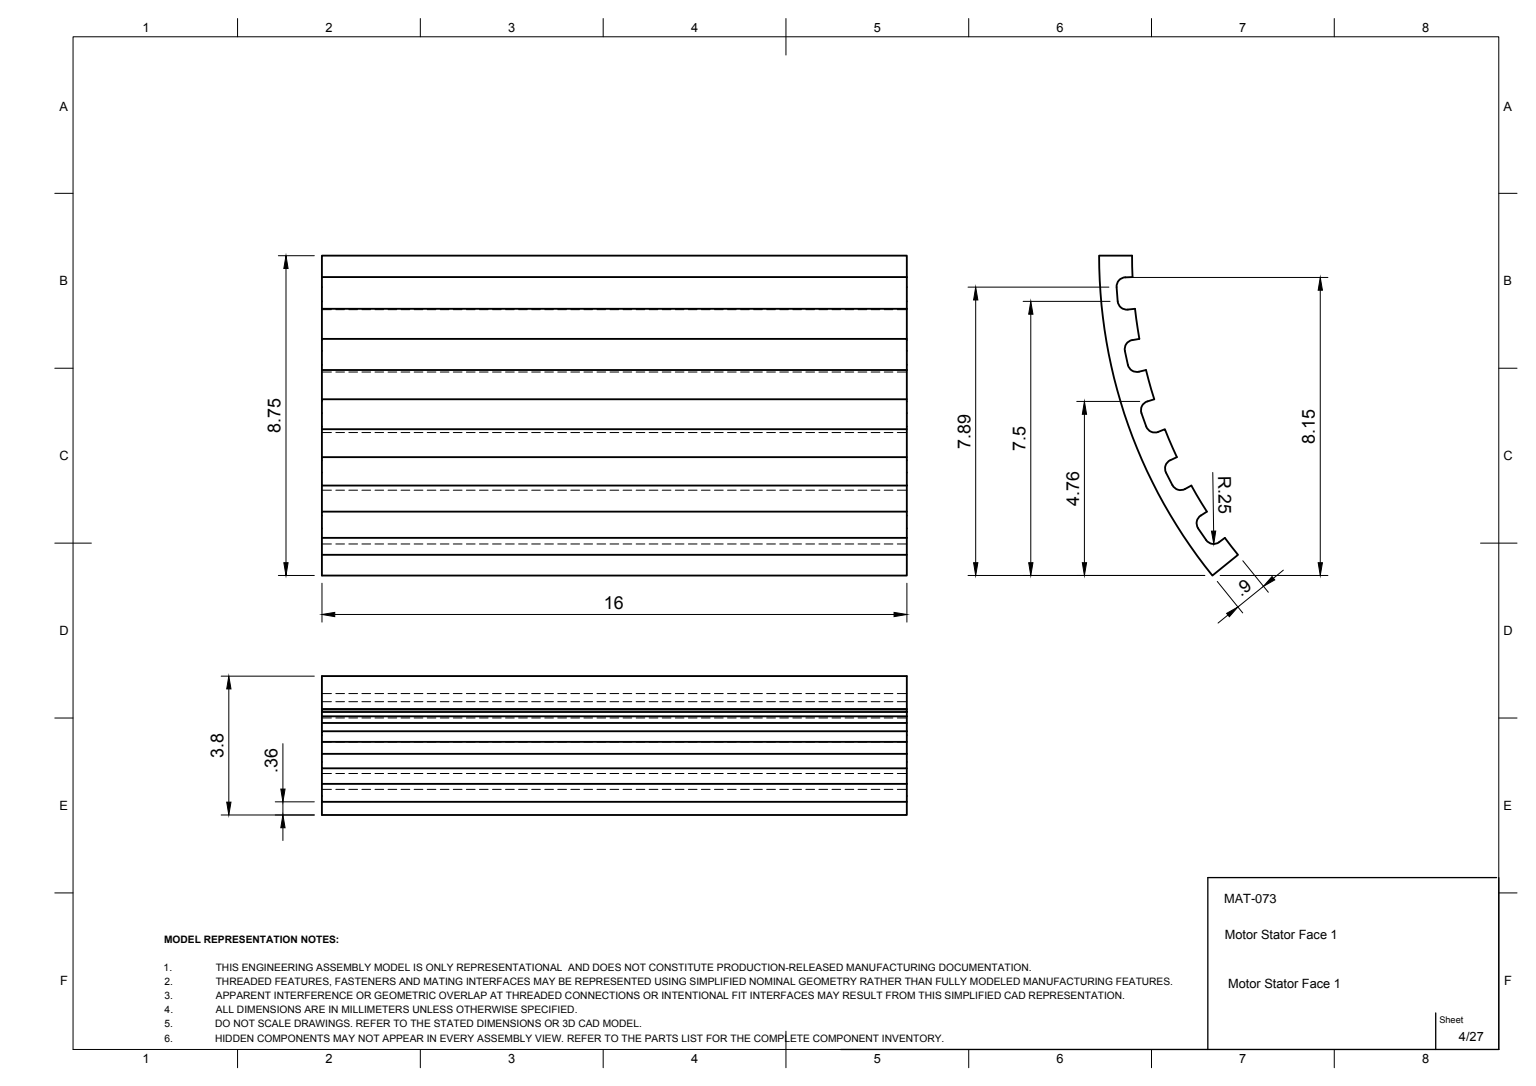
ISO-10303-21;
HEADER;
/* Generated by software containing ST-Developer
 * from STEP Tools, Inc. (www.steptools.com) 
 */

FILE_DESCRIPTION(
/* description */ ('CAx-IF Rec.Pracs.---Representation and Presentation of Product Manufa
cturing Information (PMI)---4.0---2014-10-13'),
/* implementation_level */ '2;1');

FILE_NAME(
/* name */ 'Motor Stator Face 1.step',
/* time_stamp */ '2026-10-24T18:52:33-07:00',
/* author */ (''),
/* organization */ (''),
/* preprocessor_version */ 'ST-DEVELOPER v20.2',
/* originating_system */ 'Autodesk Translation Framework v15.17.0.0',
/* authorisation */ '');

FILE_SCHEMA (('AP242_MANAGED_MODEL_BASED_3D_ENGINEERING_MIM_LF { 1 0 10303 442 2 1 4 }'));
ENDSEC;

DATA;
#10=MECHANICAL_DESIGN_GEOMETRIC_PRESENTATION_REPRESENTATION('',(#415),#34876);
#349=SHAPE_REPRESENTATION_RELATIONSHIP('SRR','None',#34986,#382);
#382=ADVANCED_BREP_SHAPE_REPRESENTATION('',(#448),#34844);
#415=STYLED_ITEM('',(#35160),#448);
#448=MANIFOLD_SOLID_BREP('Motor Stator Face 1',#19555);
#592=PLANE('',#19979);
#593=PLANE('',#19989);
#594=PLANE('',#19999);
#595=PLANE('',#20009);
#596=PLANE('',#20019);
#597=PLANE('',#20020);
#598=PLANE('',#20021);
#599=PLANE('',#20022);
#600=PLANE('',#20023);
#601=PLANE('',#20030);
#602=PLANE('',#20040);
#603=PLANE('',#20045);
#604=PLANE('',#20048);
#605=PLANE('',#20049);
#1085=LINE('',#28505,#2684);
#1086=LINE('',#28508,#2685);
#1087=LINE('',#28513,#2686);
#1088=LINE('',#28519,#2687);
#1089=LINE('',#28523,#2688);
#1090=LINE('',#28525,#2689);
#1091=LINE('',#28526,#2690);
#1092=LINE('',#28532,#2691);
#1093=LINE('',#28535,#2692);
#1094=LINE('',#28540,#2693);
#1095=LINE('',#28546,#2694);
#1096=LINE('',#28550,#2695);
#1097=LINE('',#28552,#2696);
#1098=LINE('',#28553,#2697);
#1099=LINE('',#28559,#2698);
#1100=LINE('',#28562,#2699);
#1101=LINE('',#28567,#2700);
#1102=LINE('',#28573,#2701);
#1103=LINE('',#28577,#2702);
#1104=LINE('',#28579,#2703);
#1105=LINE('',#28580,#2704);
#1106=LINE('',#28586,#2705);
#1107=LINE('',#28589,#2706);
#1108=LINE('',#28594,#2707);
#1109=LINE('',#28600,#2708);
#1110=LINE('',#28604,#2709);
#1111=LINE('',#28606,#2710);
#1112=LINE('',#28607,#2711);
#1113=LINE('',#28613,#2712);
#1114=LINE('',#28616,#2713);
#1115=LINE('',#28621,#2714);
#1116=LINE('',#28627,#2715);
#1117=LINE('',#28631,#2716);
#1118=LINE('',#28633,#2717);
#1119=LINE('',#28634,#2718);
#1120=LINE('',#28637,#2719);
#1121=LINE('',#28639,#2720);
#1122=LINE('',#28640,#2721);
#1123=LINE('',#28643,#2722);
#1124=LINE('',#28645,#2723);
#1125=LINE('',#28646,#2724);
#1126=LINE('',#28649,#2725);
#1127=LINE('',#28651,#2726);
#1128=LINE('',#28652,#2727);
#1129=LINE('',#28655,#2728);
#1130=LINE('',#28657,#2729);
#1131=LINE('',#28658,#2730);
#1132=LINE('',#28663,#2731);
#1133=LINE('',#28670,#2732);
#1134=LINE('',#28674,#2733);
#1135=LINE('',#28679,#2734);
#1136=LINE('',#28684,#2735);
#1137=LINE('',#28687,#2736);
#1138=LINE('',#28690,#2737);
#1139=LINE('',#28695,#2738);
#1140=LINE('',#28698,#2739);
#1141=LINE('',#28700,#2740);
#1142=LINE('',#28704,#2741);
#2684=VECTOR('',#22302,1.);
#2685=VECTOR('',#22305,1.);
#2686=VECTOR('',#22310,1.);
#2687=VECTOR('',#22317,1.);
#2688=VECTOR('',#22322,1.);
#2689=VECTOR('',#22323,1.);
#2690=VECTOR('',#22324,1.);
#2691=VECTOR('',#22329,1.);
#2692=VECTOR('',#22332,1.);
#2693=VECTOR('',#22337,1.);
#2694=VECTOR('',#22344,1.);
#2695=VECTOR('',#22349,0.999999999999999);
#2696=VECTOR('',#22350,1.);
#2697=VECTOR('',#22351,0.999999999999999);
#2698=VECTOR('',#22356,1.);
#2699=VECTOR('',#22359,1.);
#2700=VECTOR('',#22364,1.);
#2701=VECTOR('',#22371,1.);
#2702=VECTOR('',#22376,1.);
#2703=VECTOR('',#22377,1.);
#2704=VECTOR('',#22378,1.);
#2705=VECTOR('',#22383,1.);
#2706=VECTOR('',#22386,1.);
#2707=VECTOR('',#22391,1.);
#2708=VECTOR('',#22398,1.);
#2709=VECTOR('',#22403,1.);
#2710=VECTOR('',#22404,1.);
#2711=VECTOR('',#22405,1.);
#2712=VECTOR('',#22410,1.);
#2713=VECTOR('',#22413,1.);
#2714=VECTOR('',#22418,1.);
#2715=VECTOR('',#22425,1.);
#2716=VECTOR('',#22430,1.);
#2717=VECTOR('',#22431,1.);
#2718=VECTOR('',#22432,1.);
#2719=VECTOR('',#22435,1.);
#2720=VECTOR('',#22436,1.);
#2721=VECTOR('',#22437,1.);
#2722=VECTOR('',#22440,0.999999999999999);
#2723=VECTOR('',#22441,1.);
#2724=VECTOR('',#22442,0.999999999999999);
#2725=VECTOR('',#22445,1.);
#2726=VECTOR('',#22446,1.);
#2727=VECTOR('',#22447,1.);
#2728=VECTOR('',#22450,1.);
#2729=VECTOR('',#22451,1.);
#2730=VECTOR('',#22452,1.);
#2731=VECTOR('',#22457,1.);
#2732=VECTOR('',#22468,1.);
#2733=VECTOR('',#22471,1.);
#2734=VECTOR('',#22478,1.);
#2735=VECTOR('',#22485,1.);
#2736=VECTOR('',#22488,1.);
#2737=VECTOR('',#22493,1.);
#2738=VECTOR('',#22500,1.);
#2739=VECTOR('',#22503,1.);
#2740=VECTOR('',#22506,1.);
#2741=VECTOR('',#22513,1.);
#4283=CYLINDRICAL_SURFACE('',#19970,0.00025);
#4284=CYLINDRICAL_SURFACE('',#19973,0.01345);
#4285=CYLINDRICAL_SURFACE('',#19976,0.00025);
#4286=CYLINDRICAL_SURFACE('',#19980,0.00025);
#4287=CYLINDRICAL_SURFACE('',#19983,0.01345);
#4288=CYLINDRICAL_SURFACE('',#19986,0.00025);
#4289=CYLINDRICAL_SURFACE('',#19990,0.00025);
#4290=CYLINDRICAL_SURFACE('',#19993,0.01345);
#4291=CYLINDRICAL_SURFACE('',#19996,0.00025);
#4292=CYLINDRICAL_SURFACE('',#20000,0.00025);
#4293=CYLINDRICAL_SURFACE('',#20003,0.01345);
#4294=CYLINDRICAL_SURFACE('',#20006,0.00025);
#4295=CYLINDRICAL_SURFACE('',#20010,0.00025);
#4296=CYLINDRICAL_SURFACE('',#20013,0.01345);
#4297=CYLINDRICAL_SURFACE('',#20016,0.00025);
#4298=CYLINDRICAL_SURFACE('',#20024,0.013);
#4299=CYLINDRICAL_SURFACE('',#20027,0.013);
#4300=CYLINDRICAL_SURFACE('',#20036,0.013);
#4301=CYLINDRICAL_SURFACE('',#20038,0.013);
#4302=CYLINDRICAL_SURFACE('',#20041,0.013);
#4303=CYLINDRICAL_SURFACE('',#20043,0.0139);
#4304=CYLINDRICAL_SURFACE('',#20046,0.013);
#4799=FACE_OUTER_BOUND('',#5846,.T.);
#4800=FACE_OUTER_BOUND('',#5847,.T.);
#4801=FACE_OUTER_BOUND('',#5848,.T.);
#4802=FACE_OUTER_BOUND('',#5849,.T.);
#4803=FACE_OUTER_BOUND('',#5850,.T.);
#4804=FACE_OUTER_BOUND('',#5851,.T.);
#4805=FACE_OUTER_BOUND('',#5852,.T.);
#4806=FACE_OUTER_BOUND('',#5853,.T.);
#4807=FACE_OUTER_BOUND('',#5854,.T.);
#4808=FACE_OUTER_BOUND('',#5855,.T.);
#4809=FACE_OUTER_BOUND('',#5856,.T.);
#4810=FACE_OUTER_BOUND('',#5857,.T.);
#4811=FACE_OUTER_BOUND('',#5858,.T.);
#4812=FACE_OUTER_BOUND('',#5859,.T.);
#4813=FACE_OUTER_BOUND('',#5860,.T.);
#4814=FACE_OUTER_BOUND('',#5861,.T.);
#4815=FACE_OUTER_BOUND('',#5862,.T.);
#4816=FACE_OUTER_BOUND('',#5863,.T.);
#4817=FACE_OUTER_BOUND('',#5864,.T.);
#4818=FACE_OUTER_BOUND('',#5865,.T.);
#4819=FACE_OUTER_BOUND('',#5866,.T.);
#4820=FACE_OUTER_BOUND('',#5867,.T.);
#4821=FACE_OUTER_BOUND('',#5868,.T.);
#4822=FACE_OUTER_BOUND('',#5869,.T.);
#4823=FACE_OUTER_BOUND('',#5870,.T.);
#4824=FACE_OUTER_BOUND('',#5871,.T.);
#4825=FACE_OUTER_BOUND('',#5872,.T.);
#4826=FACE_OUTER_BOUND('',#5873,.T.);
#4827=FACE_OUTER_BOUND('',#5874,.T.);
#4828=FACE_OUTER_BOUND('',#5875,.T.);
#4829=FACE_OUTER_BOUND('',#5876,.T.);
#4830=FACE_OUTER_BOUND('',#5877,.T.);
#4831=FACE_OUTER_BOUND('',#5878,.T.);
#4832=FACE_OUTER_BOUND('',#5879,.T.);
#4833=FACE_OUTER_BOUND('',#5880,.T.);
#4834=FACE_OUTER_BOUND('',#5881,.T.);
#5846=EDGE_LOOP('',(#12830,#12831,#12832,#12833));
#5847=EDGE_LOOP('',(#12834,#12835,#12836,#12837));
#5848=EDGE_LOOP('',(#12838,#12839,#12840,#12841));
#5849=EDGE_LOOP('',(#12842,#12843,#12844,#12845));
#5850=EDGE_LOOP('',(#12846,#12847,#12848,#12849));
#5851=EDGE_LOOP('',(#12850,#12851,#12852,#12853));
#5852=EDGE_LOOP('',(#12854,#12855,#12856,#12857));
#5853=EDGE_LOOP('',(#12858,#12859,#12860,#12861));
#5854=EDGE_LOOP('',(#12862,#12863,#12864,#12865));
#5855=EDGE_LOOP('',(#12866,#12867,#12868,#12869));
#5856=EDGE_LOOP('',(#12870,#12871,#12872,#12873));
#5857=EDGE_LOOP('',(#12874,#12875,#12876,#12877));
#5858=EDGE_LOOP('',(#12878,#12879,#12880,#12881));
#5859=EDGE_LOOP('',(#12882,#12883,#12884,#12885));
#5860=EDGE_LOOP('',(#12886,#12887,#12888,#12889));
#5861=EDGE_LOOP('',(#12890,#12891,#12892,#12893));
#5862=EDGE_LOOP('',(#12894,#12895,#12896,#12897));
#5863=EDGE_LOOP('',(#12898,#12899,#12900,#12901));
#5864=EDGE_LOOP('',(#12902,#12903,#12904,#12905));
#5865=EDGE_LOOP('',(#12906,#12907,#12908,#12909));
#5866=EDGE_LOOP('',(#12910,#12911,#12912,#12913));
#5867=EDGE_LOOP('',(#12914,#12915,#12916,#12917));
#5868=EDGE_LOOP('',(#12918,#12919,#12920,#12921));
#5869=EDGE_LOOP('',(#12922,#12923,#12924,#12925));
#5870=EDGE_LOOP('',(#12926,#12927,#12928,#12929));
#5871=EDGE_LOOP('',(#12930,#12931,#12932,#12933));
#5872=EDGE_LOOP('',(#12934,#12935,#12936,#12937,#12938,#12939,#12940,#12941,
#12942,#12943,#12944,#12945,#12946,#12947,#12948,#12949,#12950,#12951,#12952,
#12953,#12954,#12955,#12956,#12957,#12958,#12959,#12960,#12961,#12962,#12963,
#12964,#12965,#12966,#12967));
#5873=EDGE_LOOP('',(#12968,#12969,#12970,#12971));
#5874=EDGE_LOOP('',(#12972,#12973,#12974,#12975));
#5875=EDGE_LOOP('',(#12976,#12977,#12978,#12979));
#5876=EDGE_LOOP('',(#12980,#12981,#12982,#12983));
#5877=EDGE_LOOP('',(#12984,#12985,#12986,#12987));
#5878=EDGE_LOOP('',(#12988,#12989,#12990,#12991));
#5879=EDGE_LOOP('',(#12992,#12993,#12994,#12995));
#5880=EDGE_LOOP('',(#12996,#12997,#12998,#12999));
#5881=EDGE_LOOP('',(#13000,#13001,#13002,#13003,#13004,#13005,#13006,#13007,
#13008,#13009,#13010,#13011,#13012,#13013,#13014,#13015,#13016,#13017,#13018,
#13019,#13020,#13021,#13022,#13023,#13024,#13025,#13026,#13027,#13028,#13029,
#13030,#13031,#13032,#13033));
#7003=CIRCLE('',#19971,0.000250000000012414);
#7004=CIRCLE('',#19972,0.000250000000012414);
#7005=CIRCLE('',#19974,0.0134500000000135);
#7006=CIRCLE('',#19975,0.0134500000000135);
#7007=CIRCLE('',#19977,0.000250000000012074);
#7008=CIRCLE('',#19978,0.000250000000012074);
#7009=CIRCLE('',#19981,0.000250000000011423);
#7010=CIRCLE('',#19982,0.000250000000011423);
#7011=CIRCLE('',#19984,0.0134500000000139);
#7012=CIRCLE('',#19985,0.0134500000000139);
#7013=CIRCLE('',#19987,0.00025000000001101);
#7014=CIRCLE('',#19988,0.00025000000001101);
#7015=CIRCLE('',#19991,0.000250000000010237);
#7016=CIRCLE('',#19992,0.000250000000010237);
#7017=CIRCLE('',#19994,0.0134500000000141);
#7018=CIRCLE('',#19995,0.0134500000000141);
#7019=CIRCLE('',#19997,0.000250000000010237);
#7020=CIRCLE('',#19998,0.000250000000010237);
#7021=CIRCLE('',#20001,0.00025000000001101);
#7022=CIRCLE('',#20002,0.00025000000001101);
#7023=CIRCLE('',#20004,0.0134500000000141);
#7024=CIRCLE('',#20005,0.0134500000000141);
#7025=CIRCLE('',#20007,0.000250000000011423);
#7026=CIRCLE('',#20008,0.000250000000011423);
#7027=CIRCLE('',#20011,0.000250000000012074);
#7028=CIRCLE('',#20012,0.000250000000012074);
#7029=CIRCLE('',#20014,0.0134500000000138);
#7030=CIRCLE('',#20015,0.0134500000000138);
#7031=CIRCLE('',#20017,0.000250000000012414);
#7032=CIRCLE('',#20018,0.000250000000012414);
#7033=CIRCLE('',#20025,0.0130000000000133);
#7034=CIRCLE('',#20026,0.0130000000000133);
#7035=CIRCLE('',#20028,0.0130000000000133);
#7036=CIRCLE('',#20029,0.0130000000000133);
#7037=CIRCLE('',#20031,0.0139000000000133);
#7038=CIRCLE('',#20032,0.0130000000000133);
#7039=CIRCLE('',#20033,0.0130000000000133);
#7040=CIRCLE('',#20034,0.0130000000000133);
#7041=CIRCLE('',#20035,0.0130000000000133);
#7042=CIRCLE('',#20037,0.0130000000000133);
#7043=CIRCLE('',#20039,0.0130000000000133);
#7044=CIRCLE('',#20042,0.0130000000000133);
#7045=CIRCLE('',#20044,0.0139000000000133);
#7046=CIRCLE('',#20047,0.0130000000000133);
#8081=VERTEX_POINT('',#28501);
#8082=VERTEX_POINT('',#28502);
#8083=VERTEX_POINT('',#28504);
#8084=VERTEX_POINT('',#28506);
#8085=VERTEX_POINT('',#28510);
#8086=VERTEX_POINT('',#28512);
#8087=VERTEX_POINT('',#28516);
#8088=VERTEX_POINT('',#28518);
#8089=VERTEX_POINT('',#28522);
#8090=VERTEX_POINT('',#28524);
#8091=VERTEX_POINT('',#28528);
#8092=VERTEX_POINT('',#28529);
#8093=VERTEX_POINT('',#28531);
#8094=VERTEX_POINT('',#28533);
#8095=VERTEX_POINT('',#28537);
#8096=VERTEX_POINT('',#28539);
#8097=VERTEX_POINT('',#28543);
#8098=VERTEX_POINT('',#28545);
#8099=VERTEX_POINT('',#28549);
#8100=VERTEX_POINT('',#28551);
#8101=VERTEX_POINT('',#28555);
#8102=VERTEX_POINT('',#28556);
#8103=VERTEX_POINT('',#28558);
#8104=VERTEX_POINT('',#28560);
#8105=VERTEX_POINT('',#28564);
#8106=VERTEX_POINT('',#28566);
#8107=VERTEX_POINT('',#28570);
#8108=VERTEX_POINT('',#28572);
#8109=VERTEX_POINT('',#28576);
#8110=VERTEX_POINT('',#28578);
#8111=VERTEX_POINT('',#28582);
#8112=VERTEX_POINT('',#28583);
#8113=VERTEX_POINT('',#28585);
#8114=VERTEX_POINT('',#28587);
#8115=VERTEX_POINT('',#28591);
#8116=VERTEX_POINT('',#28593);
#8117=VERTEX_POINT('',#28597);
#8118=VERTEX_POINT('',#28599);
#8119=VERTEX_POINT('',#28603);
#8120=VERTEX_POINT('',#28605);
#8121=VERTEX_POINT('',#28609);
#8122=VERTEX_POINT('',#28610);
#8123=VERTEX_POINT('',#28612);
#8124=VERTEX_POINT('',#28614);
#8125=VERTEX_POINT('',#28618);
#8126=VERTEX_POINT('',#28620);
#8127=VERTEX_POINT('',#28624);
#8128=VERTEX_POINT('',#28626);
#8129=VERTEX_POINT('',#28630);
#8130=VERTEX_POINT('',#28632);
#8131=VERTEX_POINT('',#28636);
#8132=VERTEX_POINT('',#28638);
#8133=VERTEX_POINT('',#28642);
#8134=VERTEX_POINT('',#28644);
#8135=VERTEX_POINT('',#28648);
#8136=VERTEX_POINT('',#28650);
#8137=VERTEX_POINT('',#28654);
#8138=VERTEX_POINT('',#28656);
#8139=VERTEX_POINT('',#28660);
#8140=VERTEX_POINT('',#28662);
#8141=VERTEX_POINT('',#28669);
#8142=VERTEX_POINT('',#28671);
#8143=VERTEX_POINT('',#28673);
#8144=VERTEX_POINT('',#28677);
#8145=VERTEX_POINT('',#28682);
#8146=VERTEX_POINT('',#28686);
#8147=VERTEX_POINT('',#28694);
#8148=VERTEX_POINT('',#28696);
#9973=EDGE_CURVE('',#8081,#8082,#7003,.T.);
#9974=EDGE_CURVE('',#8082,#8083,#1085,.T.);
#9975=EDGE_CURVE('',#8083,#8084,#7004,.T.);
#9976=EDGE_CURVE('',#8084,#8081,#1086,.T.);
#9977=EDGE_CURVE('',#8085,#8082,#7005,.T.);
#9978=EDGE_CURVE('',#8086,#8085,#1087,.T.);
#9979=EDGE_CURVE('',#8083,#8086,#7006,.T.);
#9980=EDGE_CURVE('',#8085,#8087,#7007,.T.);
#9981=EDGE_CURVE('',#8087,#8088,#1088,.T.);
#9982=EDGE_CURVE('',#8088,#8086,#7008,.T.);
#9983=EDGE_CURVE('',#8089,#8087,#1089,.T.);
#9984=EDGE_CURVE('',#8090,#8089,#1090,.T.);
#9985=EDGE_CURVE('',#8088,#8090,#1091,.T.);
#9986=EDGE_CURVE('',#8091,#8092,#7009,.T.);
#9987=EDGE_CURVE('',#8092,#8093,#1092,.T.);
#9988=EDGE_CURVE('',#8093,#8094,#7010,.T.);
#9989=EDGE_CURVE('',#8094,#8091,#1093,.T.);
#9990=EDGE_CURVE('',#8095,#8092,#7011,.T.);
#9991=EDGE_CURVE('',#8096,#8095,#1094,.T.);
#9992=EDGE_CURVE('',#8093,#8096,#7012,.T.);
#9993=EDGE_CURVE('',#8095,#8097,#7013,.T.);
#9994=EDGE_CURVE('',#8097,#8098,#1095,.T.);
#9995=EDGE_CURVE('',#8098,#8096,#7014,.T.);
#9996=EDGE_CURVE('',#8099,#8097,#1096,.T.);
#9997=EDGE_CURVE('',#8100,#8099,#1097,.T.);
#9998=EDGE_CURVE('',#8098,#8100,#1098,.T.);
#9999=EDGE_CURVE('',#8101,#8102,#7015,.T.);
#10000=EDGE_CURVE('',#8102,#8103,#1099,.T.);
#10001=EDGE_CURVE('',#8103,#8104,#7016,.T.);
#10002=EDGE_CURVE('',#8104,#8101,#1100,.T.);
#10003=EDGE_CURVE('',#8105,#8102,#7017,.T.);
#10004=EDGE_CURVE('',#8106,#8105,#1101,.T.);
#10005=EDGE_CURVE('',#8103,#8106,#7018,.T.);
#10006=EDGE_CURVE('',#8105,#8107,#7019,.T.);
#10007=EDGE_CURVE('',#8107,#8108,#1102,.T.);
#10008=EDGE_CURVE('',#8108,#8106,#7020,.T.);
#10009=EDGE_CURVE('',#8109,#8107,#1103,.T.);
#10010=EDGE_CURVE('',#8110,#8109,#1104,.T.);
#10011=EDGE_CURVE('',#8108,#8110,#1105,.T.);
#10012=EDGE_CURVE('',#8111,#8112,#7021,.T.);
#10013=EDGE_CURVE('',#8112,#8113,#1106,.T.);
#10014=EDGE_CURVE('',#8113,#8114,#7022,.T.);
#10015=EDGE_CURVE('',#8114,#8111,#1107,.T.);
#10016=EDGE_CURVE('',#8115,#8112,#7023,.T.);
#10017=EDGE_CURVE('',#8116,#8115,#1108,.T.);
#10018=EDGE_CURVE('',#8113,#8116,#7024,.T.);
#10019=EDGE_CURVE('',#8115,#8117,#7025,.T.);
#10020=EDGE_CURVE('',#8117,#8118,#1109,.T.);
#10021=EDGE_CURVE('',#8118,#8116,#7026,.T.);
#10022=EDGE_CURVE('',#8119,#8117,#1110,.T.);
#10023=EDGE_CURVE('',#8120,#8119,#1111,.T.);
#10024=EDGE_CURVE('',#8118,#8120,#1112,.T.);
#10025=EDGE_CURVE('',#8121,#8122,#7027,.T.);
#10026=EDGE_CURVE('',#8122,#8123,#1113,.T.);
#10027=EDGE_CURVE('',#8123,#8124,#7028,.T.);
#10028=EDGE_CURVE('',#8124,#8121,#1114,.T.);
#10029=EDGE_CURVE('',#8125,#8122,#7029,.T.);
#10030=EDGE_CURVE('',#8126,#8125,#1115,.T.);
#10031=EDGE_CURVE('',#8123,#8126,#7030,.T.);
#10032=EDGE_CURVE('',#8125,#8127,#7031,.T.);
#10033=EDGE_CURVE('',#8127,#8128,#1116,.T.);
#10034=EDGE_CURVE('',#8128,#8126,#7032,.T.);
#10035=EDGE_CURVE('',#8129,#8127,#1117,.T.);
#10036=EDGE_CURVE('',#8130,#8129,#1118,.T.);
#10037=EDGE_CURVE('',#8128,#8130,#1119,.T.);
#10038=EDGE_CURVE('',#8131,#8124,#1120,.T.);
#10039=EDGE_CURVE('',#8132,#8131,#1121,.T.);
#10040=EDGE_CURVE('',#8121,#8132,#1122,.T.);
#10041=EDGE_CURVE('',#8133,#8114,#1123,.T.);
#10042=EDGE_CURVE('',#8134,#8133,#1124,.T.);
#10043=EDGE_CURVE('',#8111,#8134,#1125,.T.);
#10044=EDGE_CURVE('',#8135,#8094,#1126,.T.);
#10045=EDGE_CURVE('',#8136,#8135,#1127,.T.);
#10046=EDGE_CURVE('',#8091,#8136,#1128,.T.);
#10047=EDGE_CURVE('',#8137,#8084,#1129,.T.);
#10048=EDGE_CURVE('',#8138,#8137,#1130,.T.);
#10049=EDGE_CURVE('',#8081,#8138,#1131,.T.);
#10050=EDGE_CURVE('',#8139,#8129,#7033,.T.);
#10051=EDGE_CURVE('',#8140,#8139,#1132,.T.);
#10052=EDGE_CURVE('',#8130,#8140,#7034,.T.);
#10053=EDGE_CURVE('',#8110,#8133,#7035,.T.);
#10054=EDGE_CURVE('',#8134,#8109,#7036,.T.);
#10055=EDGE_CURVE('',#8140,#8141,#1133,.T.);
#10056=EDGE_CURVE('',#8141,#8142,#7037,.T.);
#10057=EDGE_CURVE('',#8142,#8143,#1134,.T.);
#10058=EDGE_CURVE('',#8143,#8137,#7038,.T.);
#10059=EDGE_CURVE('',#8090,#8135,#7039,.T.);
#10060=EDGE_CURVE('',#8100,#8144,#7040,.T.);
#10061=EDGE_CURVE('',#8144,#8104,#1135,.T.);
#10062=EDGE_CURVE('',#8120,#8131,#7041,.T.);
#10063=EDGE_CURVE('',#8145,#8099,#7042,.T.);
#10064=EDGE_CURVE('',#8145,#8144,#1136,.T.);
#10065=EDGE_CURVE('',#8143,#8146,#1137,.T.);
#10066=EDGE_CURVE('',#8138,#8146,#7043,.T.);
#10067=EDGE_CURVE('',#8101,#8145,#1138,.T.);
#10068=EDGE_CURVE('',#8132,#8119,#7044,.T.);
#10069=EDGE_CURVE('',#8147,#8141,#1139,.T.);
#10070=EDGE_CURVE('',#8148,#8147,#7045,.T.);
#10071=EDGE_CURVE('',#8142,#8148,#1140,.T.);
#10072=EDGE_CURVE('',#8146,#8148,#1141,.T.);
#10073=EDGE_CURVE('',#8136,#8089,#7046,.T.);
#10074=EDGE_CURVE('',#8147,#8139,#1142,.T.);
#12830=ORIENTED_EDGE('',*,*,#9973,.T.);
#12831=ORIENTED_EDGE('',*,*,#9974,.T.);
#12832=ORIENTED_EDGE('',*,*,#9975,.T.);
#12833=ORIENTED_EDGE('',*,*,#9976,.T.);
#12834=ORIENTED_EDGE('',*,*,#9974,.F.);
#12835=ORIENTED_EDGE('',*,*,#9977,.F.);
#12836=ORIENTED_EDGE('',*,*,#9978,.F.);
#12837=ORIENTED_EDGE('',*,*,#9979,.F.);
#12838=ORIENTED_EDGE('',*,*,#9980,.T.);
#12839=ORIENTED_EDGE('',*,*,#9981,.T.);
#12840=ORIENTED_EDGE('',*,*,#9982,.T.);
#12841=ORIENTED_EDGE('',*,*,#9978,.T.);
#12842=ORIENTED_EDGE('',*,*,#9981,.F.);
#12843=ORIENTED_EDGE('',*,*,#9983,.F.);
#12844=ORIENTED_EDGE('',*,*,#9984,.F.);
#12845=ORIENTED_EDGE('',*,*,#9985,.F.);
#12846=ORIENTED_EDGE('',*,*,#9986,.T.);
#12847=ORIENTED_EDGE('',*,*,#9987,.T.);
#12848=ORIENTED_EDGE('',*,*,#9988,.T.);
#12849=ORIENTED_EDGE('',*,*,#9989,.T.);
#12850=ORIENTED_EDGE('',*,*,#9987,.F.);
#12851=ORIENTED_EDGE('',*,*,#9990,.F.);
#12852=ORIENTED_EDGE('',*,*,#9991,.F.);
#12853=ORIENTED_EDGE('',*,*,#9992,.F.);
#12854=ORIENTED_EDGE('',*,*,#9993,.T.);
#12855=ORIENTED_EDGE('',*,*,#9994,.T.);
#12856=ORIENTED_EDGE('',*,*,#9995,.T.);
#12857=ORIENTED_EDGE('',*,*,#9991,.T.);
#12858=ORIENTED_EDGE('',*,*,#9994,.F.);
#12859=ORIENTED_EDGE('',*,*,#9996,.F.);
#12860=ORIENTED_EDGE('',*,*,#9997,.F.);
#12861=ORIENTED_EDGE('',*,*,#9998,.F.);
#12862=ORIENTED_EDGE('',*,*,#9999,.T.);
#12863=ORIENTED_EDGE('',*,*,#10000,.T.);
#12864=ORIENTED_EDGE('',*,*,#10001,.T.);
#12865=ORIENTED_EDGE('',*,*,#10002,.T.);
#12866=ORIENTED_EDGE('',*,*,#10000,.F.);
#12867=ORIENTED_EDGE('',*,*,#10003,.F.);
#12868=ORIENTED_EDGE('',*,*,#10004,.F.);
#12869=ORIENTED_EDGE('',*,*,#10005,.F.);
#12870=ORIENTED_EDGE('',*,*,#10006,.T.);
#12871=ORIENTED_EDGE('',*,*,#10007,.T.);
#12872=ORIENTED_EDGE('',*,*,#10008,.T.);
#12873=ORIENTED_EDGE('',*,*,#10004,.T.);
#12874=ORIENTED_EDGE('',*,*,#10007,.F.);
#12875=ORIENTED_EDGE('',*,*,#10009,.F.);
#12876=ORIENTED_EDGE('',*,*,#10010,.F.);
#12877=ORIENTED_EDGE('',*,*,#10011,.F.);
#12878=ORIENTED_EDGE('',*,*,#10012,.T.);
#12879=ORIENTED_EDGE('',*,*,#10013,.T.);
#12880=ORIENTED_EDGE('',*,*,#10014,.T.);
#12881=ORIENTED_EDGE('',*,*,#10015,.T.);
#12882=ORIENTED_EDGE('',*,*,#10013,.F.);
#12883=ORIENTED_EDGE('',*,*,#10016,.F.);
#12884=ORIENTED_EDGE('',*,*,#10017,.F.);
#12885=ORIENTED_EDGE('',*,*,#10018,.F.);
#12886=ORIENTED_EDGE('',*,*,#10019,.T.);
#12887=ORIENTED_EDGE('',*,*,#10020,.T.);
#12888=ORIENTED_EDGE('',*,*,#10021,.T.);
#12889=ORIENTED_EDGE('',*,*,#10017,.T.);
#12890=ORIENTED_EDGE('',*,*,#10020,.F.);
#12891=ORIENTED_EDGE('',*,*,#10022,.F.);
#12892=ORIENTED_EDGE('',*,*,#10023,.F.);
#12893=ORIENTED_EDGE('',*,*,#10024,.F.);
#12894=ORIENTED_EDGE('',*,*,#10025,.T.);
#12895=ORIENTED_EDGE('',*,*,#10026,.T.);
#12896=ORIENTED_EDGE('',*,*,#10027,.T.);
#12897=ORIENTED_EDGE('',*,*,#10028,.T.);
#12898=ORIENTED_EDGE('',*,*,#10026,.F.);
#12899=ORIENTED_EDGE('',*,*,#10029,.F.);
#12900=ORIENTED_EDGE('',*,*,#10030,.F.);
#12901=ORIENTED_EDGE('',*,*,#10031,.F.);
#12902=ORIENTED_EDGE('',*,*,#10032,.T.);
#12903=ORIENTED_EDGE('',*,*,#10033,.T.);
#12904=ORIENTED_EDGE('',*,*,#10034,.T.);
#12905=ORIENTED_EDGE('',*,*,#10030,.T.);
#12906=ORIENTED_EDGE('',*,*,#10033,.F.);
#12907=ORIENTED_EDGE('',*,*,#10035,.F.);
#12908=ORIENTED_EDGE('',*,*,#10036,.F.);
#12909=ORIENTED_EDGE('',*,*,#10037,.F.);
#12910=ORIENTED_EDGE('',*,*,#10028,.F.);
#12911=ORIENTED_EDGE('',*,*,#10038,.F.);
#12912=ORIENTED_EDGE('',*,*,#10039,.F.);
#12913=ORIENTED_EDGE('',*,*,#10040,.F.);
#12914=ORIENTED_EDGE('',*,*,#10015,.F.);
#12915=ORIENTED_EDGE('',*,*,#10041,.F.);
#12916=ORIENTED_EDGE('',*,*,#10042,.F.);
#12917=ORIENTED_EDGE('',*,*,#10043,.F.);
#12918=ORIENTED_EDGE('',*,*,#9989,.F.);
#12919=ORIENTED_EDGE('',*,*,#10044,.F.);
#12920=ORIENTED_EDGE('',*,*,#10045,.F.);
#12921=ORIENTED_EDGE('',*,*,#10046,.F.);
#12922=ORIENTED_EDGE('',*,*,#9976,.F.);
#12923=ORIENTED_EDGE('',*,*,#10047,.F.);
#12924=ORIENTED_EDGE('',*,*,#10048,.F.);
#12925=ORIENTED_EDGE('',*,*,#10049,.F.);
#12926=ORIENTED_EDGE('',*,*,#10036,.T.);
#12927=ORIENTED_EDGE('',*,*,#10050,.F.);
#12928=ORIENTED_EDGE('',*,*,#10051,.F.);
#12929=ORIENTED_EDGE('',*,*,#10052,.F.);
#12930=ORIENTED_EDGE('',*,*,#10042,.T.);
#12931=ORIENTED_EDGE('',*,*,#10053,.F.);
#12932=ORIENTED_EDGE('',*,*,#10010,.T.);
#12933=ORIENTED_EDGE('',*,*,#10054,.F.);
#12934=ORIENTED_EDGE('',*,*,#10038,.T.);
#12935=ORIENTED_EDGE('',*,*,#10027,.F.);
#12936=ORIENTED_EDGE('',*,*,#10031,.T.);
#12937=ORIENTED_EDGE('',*,*,#10034,.F.);
#12938=ORIENTED_EDGE('',*,*,#10037,.T.);
#12939=ORIENTED_EDGE('',*,*,#10052,.T.);
#12940=ORIENTED_EDGE('',*,*,#10055,.T.);
#12941=ORIENTED_EDGE('',*,*,#10056,.T.);
#12942=ORIENTED_EDGE('',*,*,#10057,.T.);
#12943=ORIENTED_EDGE('',*,*,#10058,.T.);
#12944=ORIENTED_EDGE('',*,*,#10047,.T.);
#12945=ORIENTED_EDGE('',*,*,#9975,.F.);
#12946=ORIENTED_EDGE('',*,*,#9979,.T.);
#12947=ORIENTED_EDGE('',*,*,#9982,.F.);
#12948=ORIENTED_EDGE('',*,*,#9985,.T.);
#12949=ORIENTED_EDGE('',*,*,#10059,.T.);
#12950=ORIENTED_EDGE('',*,*,#10044,.T.);
#12951=ORIENTED_EDGE('',*,*,#9988,.F.);
#12952=ORIENTED_EDGE('',*,*,#9992,.T.);
#12953=ORIENTED_EDGE('',*,*,#9995,.F.);
#12954=ORIENTED_EDGE('',*,*,#9998,.T.);
#12955=ORIENTED_EDGE('',*,*,#10060,.T.);
#12956=ORIENTED_EDGE('',*,*,#10061,.T.);
#12957=ORIENTED_EDGE('',*,*,#10001,.F.);
#12958=ORIENTED_EDGE('',*,*,#10005,.T.);
#12959=ORIENTED_EDGE('',*,*,#10008,.F.);
#12960=ORIENTED_EDGE('',*,*,#10011,.T.);
#12961=ORIENTED_EDGE('',*,*,#10053,.T.);
#12962=ORIENTED_EDGE('',*,*,#10041,.T.);
#12963=ORIENTED_EDGE('',*,*,#10014,.F.);
#12964=ORIENTED_EDGE('',*,*,#10018,.T.);
#12965=ORIENTED_EDGE('',*,*,#10021,.F.);
#12966=ORIENTED_EDGE('',*,*,#10024,.T.);
#12967=ORIENTED_EDGE('',*,*,#10062,.T.);
#12968=ORIENTED_EDGE('',*,*,#9997,.T.);
#12969=ORIENTED_EDGE('',*,*,#10063,.F.);
#12970=ORIENTED_EDGE('',*,*,#10064,.T.);
#12971=ORIENTED_EDGE('',*,*,#10060,.F.);
#12972=ORIENTED_EDGE('',*,*,#10048,.T.);
#12973=ORIENTED_EDGE('',*,*,#10058,.F.);
#12974=ORIENTED_EDGE('',*,*,#10065,.T.);
#12975=ORIENTED_EDGE('',*,*,#10066,.F.);
#12976=ORIENTED_EDGE('',*,*,#10002,.F.);
#12977=ORIENTED_EDGE('',*,*,#10061,.F.);
#12978=ORIENTED_EDGE('',*,*,#10064,.F.);
#12979=ORIENTED_EDGE('',*,*,#10067,.F.);
#12980=ORIENTED_EDGE('',*,*,#10039,.T.);
#12981=ORIENTED_EDGE('',*,*,#10062,.F.);
#12982=ORIENTED_EDGE('',*,*,#10023,.T.);
#12983=ORIENTED_EDGE('',*,*,#10068,.F.);
#12984=ORIENTED_EDGE('',*,*,#10069,.F.);
#12985=ORIENTED_EDGE('',*,*,#10070,.F.);
#12986=ORIENTED_EDGE('',*,*,#10071,.F.);
#12987=ORIENTED_EDGE('',*,*,#10056,.F.);
#12988=ORIENTED_EDGE('',*,*,#10071,.T.);
#12989=ORIENTED_EDGE('',*,*,#10072,.F.);
#12990=ORIENTED_EDGE('',*,*,#10065,.F.);
#12991=ORIENTED_EDGE('',*,*,#10057,.F.);
#12992=ORIENTED_EDGE('',*,*,#10045,.T.);
#12993=ORIENTED_EDGE('',*,*,#10059,.F.);
#12994=ORIENTED_EDGE('',*,*,#9984,.T.);
#12995=ORIENTED_EDGE('',*,*,#10073,.F.);
#12996=ORIENTED_EDGE('',*,*,#10051,.T.);
#12997=ORIENTED_EDGE('',*,*,#10074,.F.);
#12998=ORIENTED_EDGE('',*,*,#10069,.T.);
#12999=ORIENTED_EDGE('',*,*,#10055,.F.);
#13000=ORIENTED_EDGE('',*,*,#10040,.T.);
#13001=ORIENTED_EDGE('',*,*,#10068,.T.);
#13002=ORIENTED_EDGE('',*,*,#10022,.T.);
#13003=ORIENTED_EDGE('',*,*,#10019,.F.);
#13004=ORIENTED_EDGE('',*,*,#10016,.T.);
#13005=ORIENTED_EDGE('',*,*,#10012,.F.);
#13006=ORIENTED_EDGE('',*,*,#10043,.T.);
#13007=ORIENTED_EDGE('',*,*,#10054,.T.);
#13008=ORIENTED_EDGE('',*,*,#10009,.T.);
#13009=ORIENTED_EDGE('',*,*,#10006,.F.);
#13010=ORIENTED_EDGE('',*,*,#10003,.T.);
#13011=ORIENTED_EDGE('',*,*,#9999,.F.);
#13012=ORIENTED_EDGE('',*,*,#10067,.T.);
#13013=ORIENTED_EDGE('',*,*,#10063,.T.);
#13014=ORIENTED_EDGE('',*,*,#9996,.T.);
#13015=ORIENTED_EDGE('',*,*,#9993,.F.);
#13016=ORIENTED_EDGE('',*,*,#9990,.T.);
#13017=ORIENTED_EDGE('',*,*,#9986,.F.);
#13018=ORIENTED_EDGE('',*,*,#10046,.T.);
#13019=ORIENTED_EDGE('',*,*,#10073,.T.);
#13020=ORIENTED_EDGE('',*,*,#9983,.T.);
#13021=ORIENTED_EDGE('',*,*,#9980,.F.);
#13022=ORIENTED_EDGE('',*,*,#9977,.T.);
#13023=ORIENTED_EDGE('',*,*,#9973,.F.);
#13024=ORIENTED_EDGE('',*,*,#10049,.T.);
#13025=ORIENTED_EDGE('',*,*,#10066,.T.);
#13026=ORIENTED_EDGE('',*,*,#10072,.T.);
#13027=ORIENTED_EDGE('',*,*,#10070,.T.);
#13028=ORIENTED_EDGE('',*,*,#10074,.T.);
#13029=ORIENTED_EDGE('',*,*,#10050,.T.);
#13030=ORIENTED_EDGE('',*,*,#10035,.T.);
#13031=ORIENTED_EDGE('',*,*,#10032,.F.);
#13032=ORIENTED_EDGE('',*,*,#10029,.T.);
#13033=ORIENTED_EDGE('',*,*,#10025,.F.);
#18515=ADVANCED_FACE('',(#4799),#4283,.F.);
#18516=ADVANCED_FACE('',(#4800),#4284,.F.);
#18517=ADVANCED_FACE('',(#4801),#4285,.F.);
#18518=ADVANCED_FACE('',(#4802),#592,.F.);
#18519=ADVANCED_FACE('',(#4803),#4286,.F.);
#18520=ADVANCED_FACE('',(#4804),#4287,.F.);
#18521=ADVANCED_FACE('',(#4805),#4288,.F.);
#18522=ADVANCED_FACE('',(#4806),#593,.F.);
#18523=ADVANCED_FACE('',(#4807),#4289,.F.);
#18524=ADVANCED_FACE('',(#4808),#4290,.F.);
#18525=ADVANCED_FACE('',(#4809),#4291,.F.);
#18526=ADVANCED_FACE('',(#4810),#594,.F.);
#18527=ADVANCED_FACE('',(#4811),#4292,.F.);
#18528=ADVANCED_FACE('',(#4812),#4293,.F.);
#18529=ADVANCED_FACE('',(#4813),#4294,.F.);
#18530=ADVANCED_FACE('',(#4814),#595,.F.);
#18531=ADVANCED_FACE('',(#4815),#4295,.F.);
#18532=ADVANCED_FACE('',(#4816),#4296,.F.);
#18533=ADVANCED_FACE('',(#4817),#4297,.F.);
#18534=ADVANCED_FACE('',(#4818),#596,.F.);
#18535=ADVANCED_FACE('',(#4819),#597,.F.);
#18536=ADVANCED_FACE('',(#4820),#598,.F.);
#18537=ADVANCED_FACE('',(#4821),#599,.F.);
#18538=ADVANCED_FACE('',(#4822),#600,.F.);
#18539=ADVANCED_FACE('',(#4823),#4298,.F.);
#18540=ADVANCED_FACE('',(#4824),#4299,.F.);
#18541=ADVANCED_FACE('',(#4825),#601,.F.);
#18542=ADVANCED_FACE('',(#4826),#4300,.F.);
#18543=ADVANCED_FACE('',(#4827),#4301,.F.);
#18544=ADVANCED_FACE('',(#4828),#602,.F.);
#18545=ADVANCED_FACE('',(#4829),#4302,.F.);
#18546=ADVANCED_FACE('',(#4830),#4303,.T.);
#18547=ADVANCED_FACE('',(#4831),#603,.T.);
#18548=ADVANCED_FACE('',(#4832),#4304,.F.);
#18549=ADVANCED_FACE('',(#4833),#604,.T.);
#18550=ADVANCED_FACE('',(#4834),#605,.T.);
#19555=CLOSED_SHELL('',(#18515,#18516,#18517,#18518,#18519,#18520,#18521,
#18522,#18523,#18524,#18525,#18526,#18527,#18528,#18529,#18530,#18531,#18532,
#18533,#18534,#18535,#18536,#18537,#18538,#18539,#18540,#18541,#18542,#18543,
#18544,#18545,#18546,#18547,#18548,#18549,#18550));
#19969=AXIS2_PLACEMENT_3D('',#28499,#22296,#22297);
#19970=AXIS2_PLACEMENT_3D('',#28500,#22298,#22299);
#19971=AXIS2_PLACEMENT_3D('',#28503,#22300,#22301);
#19972=AXIS2_PLACEMENT_3D('',#28507,#22303,#22304);
#19973=AXIS2_PLACEMENT_3D('',#28509,#22306,#22307);
#19974=AXIS2_PLACEMENT_3D('',#28511,#22308,#22309);
#19975=AXIS2_PLACEMENT_3D('',#28514,#22311,#22312);
#19976=AXIS2_PLACEMENT_3D('',#28515,#22313,#22314);
#19977=AXIS2_PLACEMENT_3D('',#28517,#22315,#22316);
#19978=AXIS2_PLACEMENT_3D('',#28520,#22318,#22319);
#19979=AXIS2_PLACEMENT_3D('',#28521,#22320,#22321);
#19980=AXIS2_PLACEMENT_3D('',#28527,#22325,#22326);
#19981=AXIS2_PLACEMENT_3D('',#28530,#22327,#22328);
#19982=AXIS2_PLACEMENT_3D('',#28534,#22330,#22331);
#19983=AXIS2_PLACEMENT_3D('',#28536,#22333,#22334);
#19984=AXIS2_PLACEMENT_3D('',#28538,#22335,#22336);
#19985=AXIS2_PLACEMENT_3D('',#28541,#22338,#22339);
#19986=AXIS2_PLACEMENT_3D('',#28542,#22340,#22341);
#19987=AXIS2_PLACEMENT_3D('',#28544,#22342,#22343);
#19988=AXIS2_PLACEMENT_3D('',#28547,#22345,#22346);
#19989=AXIS2_PLACEMENT_3D('',#28548,#22347,#22348);
#19990=AXIS2_PLACEMENT_3D('',#28554,#22352,#22353);
#19991=AXIS2_PLACEMENT_3D('',#28557,#22354,#22355);
#19992=AXIS2_PLACEMENT_3D('',#28561,#22357,#22358);
#19993=AXIS2_PLACEMENT_3D('',#28563,#22360,#22361);
#19994=AXIS2_PLACEMENT_3D('',#28565,#22362,#22363);
#19995=AXIS2_PLACEMENT_3D('',#28568,#22365,#22366);
#19996=AXIS2_PLACEMENT_3D('',#28569,#22367,#22368);
#19997=AXIS2_PLACEMENT_3D('',#28571,#22369,#22370);
#19998=AXIS2_PLACEMENT_3D('',#28574,#22372,#22373);
#19999=AXIS2_PLACEMENT_3D('',#28575,#22374,#22375);
#20000=AXIS2_PLACEMENT_3D('',#28581,#22379,#22380);
#20001=AXIS2_PLACEMENT_3D('',#28584,#22381,#22382);
#20002=AXIS2_PLACEMENT_3D('',#28588,#22384,#22385);
#20003=AXIS2_PLACEMENT_3D('',#28590,#22387,#22388);
#20004=AXIS2_PLACEMENT_3D('',#28592,#22389,#22390);
#20005=AXIS2_PLACEMENT_3D('',#28595,#22392,#22393);
#20006=AXIS2_PLACEMENT_3D('',#28596,#22394,#22395);
#20007=AXIS2_PLACEMENT_3D('',#28598,#22396,#22397);
#20008=AXIS2_PLACEMENT_3D('',#28601,#22399,#22400);
#20009=AXIS2_PLACEMENT_3D('',#28602,#22401,#22402);
#20010=AXIS2_PLACEMENT_3D('',#28608,#22406,#22407);
#20011=AXIS2_PLACEMENT_3D('',#28611,#22408,#22409);
#20012=AXIS2_PLACEMENT_3D('',#28615,#22411,#22412);
#20013=AXIS2_PLACEMENT_3D('',#28617,#22414,#22415);
#20014=AXIS2_PLACEMENT_3D('',#28619,#22416,#22417);
#20015=AXIS2_PLACEMENT_3D('',#28622,#22419,#22420);
#20016=AXIS2_PLACEMENT_3D('',#28623,#22421,#22422);
#20017=AXIS2_PLACEMENT_3D('',#28625,#22423,#22424);
#20018=AXIS2_PLACEMENT_3D('',#28628,#22426,#22427);
#20019=AXIS2_PLACEMENT_3D('',#28629,#22428,#22429);
#20020=AXIS2_PLACEMENT_3D('',#28635,#22433,#22434);
#20021=AXIS2_PLACEMENT_3D('',#28641,#22438,#22439);
#20022=AXIS2_PLACEMENT_3D('',#28647,#22443,#22444);
#20023=AXIS2_PLACEMENT_3D('',#28653,#22448,#22449);
#20024=AXIS2_PLACEMENT_3D('',#28659,#22453,#22454);
#20025=AXIS2_PLACEMENT_3D('',#28661,#22455,#22456);
#20026=AXIS2_PLACEMENT_3D('',#28664,#22458,#22459);
#20027=AXIS2_PLACEMENT_3D('',#28665,#22460,#22461);
#20028=AXIS2_PLACEMENT_3D('',#28666,#22462,#22463);
#20029=AXIS2_PLACEMENT_3D('',#28667,#22464,#22465);
#20030=AXIS2_PLACEMENT_3D('',#28668,#22466,#22467);
#20031=AXIS2_PLACEMENT_3D('',#28672,#22469,#22470);
#20032=AXIS2_PLACEMENT_3D('',#28675,#22472,#22473);
#20033=AXIS2_PLACEMENT_3D('',#28676,#22474,#22475);
#20034=AXIS2_PLACEMENT_3D('',#28678,#22476,#22477);
#20035=AXIS2_PLACEMENT_3D('',#28680,#22479,#22480);
#20036=AXIS2_PLACEMENT_3D('',#28681,#22481,#22482);
#20037=AXIS2_PLACEMENT_3D('',#28683,#22483,#22484);
#20038=AXIS2_PLACEMENT_3D('',#28685,#22486,#22487);
#20039=AXIS2_PLACEMENT_3D('',#28688,#22489,#22490);
#20040=AXIS2_PLACEMENT_3D('',#28689,#22491,#22492);
#20041=AXIS2_PLACEMENT_3D('',#28691,#22494,#22495);
#20042=AXIS2_PLACEMENT_3D('',#28692,#22496,#22497);
#20043=AXIS2_PLACEMENT_3D('',#28693,#22498,#22499);
#20044=AXIS2_PLACEMENT_3D('',#28697,#22501,#22502);
#20045=AXIS2_PLACEMENT_3D('',#28699,#22504,#22505);
#20046=AXIS2_PLACEMENT_3D('',#28701,#22507,#22508);
#20047=AXIS2_PLACEMENT_3D('',#28702,#22509,#22510);
#20048=AXIS2_PLACEMENT_3D('',#28703,#22511,#22512);
#20049=AXIS2_PLACEMENT_3D('',#28705,#22514,#22515);
#22296=DIRECTION('axis',(0.,0.,1.));
#22297=DIRECTION('refdir',(1.,0.,0.));
#22298=DIRECTION('center_axis',(0.,-1.,0.));
#22299=DIRECTION('ref_axis',(0.959438500558772,0.,0.281918008728665));
#22300=DIRECTION('center_axis',(0.,1.,0.));
#22301=DIRECTION('ref_axis',(0.959438500551132,0.,0.281918008754666));
#22302=DIRECTION('',(0.,-1.,0.));
#22303=DIRECTION('center_axis',(0.,-1.,0.));
#22304=DIRECTION('ref_axis',(0.959438500551132,0.,0.281918008754666));
#22305=DIRECTION('',(0.,1.,0.));
#22306=DIRECTION('center_axis',(0.,-1.,0.));
#22307=DIRECTION('ref_axis',(0.882269183586981,0.,-0.470745247127108));
#22308=DIRECTION('center_axis',(0.,-1.,0.));
#22309=DIRECTION('ref_axis',(0.882269183586837,0.,-0.470745247127378));
#22310=DIRECTION('',(0.,1.,0.));
#22311=DIRECTION('center_axis',(0.,1.,0.));
#22312=DIRECTION('ref_axis',(0.882269183586837,0.,-0.470745247127378));
#22313=DIRECTION('center_axis',(0.,-1.,0.));
#22314=DIRECTION('ref_axis',(0.235571092936033,0.,-0.971857119217081));
#22315=DIRECTION('center_axis',(0.,1.,0.));
#22316=DIRECTION('ref_axis',(0.235571092964656,0.,-0.971857119210143));
#22317=DIRECTION('',(0.,-1.,0.));
#22318=DIRECTION('center_axis',(0.,-1.,0.));
#22319=DIRECTION('ref_axis',(0.235571092964656,0.,-0.971857119210143));
#22320=DIRECTION('center_axis',(-0.528694902398929,0.,-0.848811934516349));
#22321=DIRECTION('ref_axis',(-0.848811934516349,0.,0.528694902398929));
#22322=DIRECTION('',(0.84881193451618,0.,-0.528694902399201));
#22323=DIRECTION('',(0.,1.,0.));
#22324=DIRECTION('',(-0.84881193451618,0.,0.528694902399201));
#22325=DIRECTION('center_axis',(0.,-1.,0.));
#22326=DIRECTION('ref_axis',(0.9880280553808,0.,0.154274306935522));
#22327=DIRECTION('center_axis',(0.,1.,0.));
#22328=DIRECTION('ref_axis',(0.988028055375654,0.,0.154274306968473));
#22329=DIRECTION('',(0.,-1.,0.));
#22330=DIRECTION('center_axis',(0.,-1.,0.));
#22331=DIRECTION('ref_axis',(0.988028055375654,0.,0.154274306968473));
#22332=DIRECTION('',(0.,1.,0.));
#22333=DIRECTION('center_axis',(0.,-1.,0.));
#22334=DIRECTION('ref_axis',(0.813276663802591,0.,-0.581877193327017));
#22335=DIRECTION('center_axis',(0.,-1.,0.));
#22336=DIRECTION('ref_axis',(0.813276663802491,0.,-0.581877193327157));
#22337=DIRECTION('',(0.,1.,0.));
#22338=DIRECTION('center_axis',(0.,1.,0.));
#22339=DIRECTION('ref_axis',(0.813276663802491,0.,-0.581877193327157));
#22340=DIRECTION('center_axis',(0.,-1.,0.));
#22341=DIRECTION('ref_axis',(0.106702940426287,0.,-0.994290944595386));
#22342=DIRECTION('center_axis',(0.,1.,0.));
#22343=DIRECTION('ref_axis',(0.106702940461588,0.,-0.994290944591597));
#22344=DIRECTION('',(0.,-1.,0.));
#22345=DIRECTION('center_axis',(0.,-1.,0.));
#22346=DIRECTION('ref_axis',(0.106702940461588,0.,-0.994290944591597));
#22347=DIRECTION('center_axis',(-0.634964033941301,0.,-0.772541698292714));
#22348=DIRECTION('ref_axis',(-0.772541698292714,0.,0.634964033941301));
#22349=DIRECTION('',(0.772541698292626,0.,-0.634964033941407));
#22350=DIRECTION('',(0.,1.,0.));
#22351=DIRECTION('',(-0.772541698292626,0.,0.634964033941407));
#22352=DIRECTION('center_axis',(0.,-1.,0.));
#22353=DIRECTION('ref_axis',(0.999712176242133,0.,0.0239909289777986));
#22354=DIRECTION('center_axis',(0.,1.,0.));
#22355=DIRECTION('ref_axis',(0.999712176241197,0.,0.0239909290168162));
#22356=DIRECTION('',(0.,-1.,0.));
#22357=DIRECTION('center_axis',(0.,-1.,0.));
#22358=DIRECTION('ref_axis',(0.999712176241197,0.,0.0239909290168162));
#22359=DIRECTION('',(0.,1.,0.));
#22360=DIRECTION('center_axis',(0.,-1.,0.));
#22361=DIRECTION('ref_axis',(0.730368754817649,0.,-0.683053059422266));
#22362=DIRECTION('center_axis',(0.,-1.,0.));
#22363=DIRECTION('ref_axis',(0.730368754817625,0.,-0.683053059422291));
#22364=DIRECTION('',(0.,1.,0.));
#22365=DIRECTION('center_axis',(0.,1.,0.));
#22366=DIRECTION('ref_axis',(0.730368754817625,0.,-0.683053059422291));
#22367=DIRECTION('center_axis',(0.,-1.,0.));
#22368=DIRECTION('ref_axis',(-0.0239909289777984,0.,-0.999712176242133));
#22369=DIRECTION('center_axis',(0.,1.,0.));
#22370=DIRECTION('ref_axis',(-0.023990929016816,0.,-0.999712176241197));
#22371=DIRECTION('',(0.,-1.,0.));
#22372=DIRECTION('center_axis',(0.,-1.,0.));
#22373=DIRECTION('ref_axis',(-0.023990929016816,0.,-0.999712176241197));
#22374=DIRECTION('center_axis',(-0.730368754817648,0.,-0.683053059422266));
#22375=DIRECTION('ref_axis',(-0.683053059422266,0.,0.730368754817648));
#22376=DIRECTION('',(0.683053059422301,0.,-0.730368754817616));
#22377=DIRECTION('',(0.,1.,0.));
#22378=DIRECTION('',(-0.683053059422301,0.,0.730368754817616));
#22379=DIRECTION('center_axis',(0.,-1.,0.));
#22380=DIRECTION('ref_axis',(0.994290944595384,0.,-0.106702940426299));
#22381=DIRECTION('center_axis',(0.,1.,0.));
#22382=DIRECTION('ref_axis',(0.994290944591596,0.,-0.1067029404616));
#22383=DIRECTION('',(0.,-1.,0.));
#22384=DIRECTION('center_axis',(0.,-1.,0.));
#22385=DIRECTION('ref_axis',(0.994290944591596,0.,-0.1067029404616));
#22386=DIRECTION('',(0.,1.,0.));
#22387=DIRECTION('center_axis',(0.,-1.,0.));
#22388=DIRECTION('ref_axis',(0.634964033941301,0.,-0.772541698292714));
#22389=DIRECTION('center_axis',(0.,-1.,0.));
#22390=DIRECTION('ref_axis',(0.63496403394138,0.,-0.772541698292649));
#22391=DIRECTION('',(0.,1.,0.));
#22392=DIRECTION('center_axis',(0.,1.,0.));
#22393=DIRECTION('ref_axis',(0.63496403394138,0.,-0.772541698292649));
#22394=DIRECTION('center_axis',(0.,-1.,0.));
#22395=DIRECTION('ref_axis',(-0.15427430693553,0.,-0.988028055380798));
#22396=DIRECTION('center_axis',(0.,1.,0.));
#22397=DIRECTION('ref_axis',(-0.154274306968481,0.,-0.988028055375653));
#22398=DIRECTION('',(0.,-1.,0.));
#22399=DIRECTION('center_axis',(0.,-1.,0.));
#22400=DIRECTION('ref_axis',(-0.154274306968481,0.,-0.988028055375653));
#22401=DIRECTION('center_axis',(-0.813276663802591,0.,-0.581877193327018));
#22402=DIRECTION('ref_axis',(-0.581877193327018,0.,0.813276663802591));
#22403=DIRECTION('',(0.581877193327206,0.,-0.813276663802456));
#22404=DIRECTION('',(0.,1.,0.));
#22405=DIRECTION('',(-0.581877193327206,0.,0.813276663802456));
#22406=DIRECTION('center_axis',(0.,-1.,0.));
#22407=DIRECTION('ref_axis',(0.971857119217081,0.,-0.235571092936033));
#22408=DIRECTION('center_axis',(0.,1.,0.));
#22409=DIRECTION('ref_axis',(0.971857119210143,0.,-0.235571092964656));
#22410=DIRECTION('',(0.,-1.,0.));
#22411=DIRECTION('center_axis',(0.,-1.,0.));
#22412=DIRECTION('ref_axis',(0.971857119210143,0.,-0.235571092964656));
#22413=DIRECTION('',(0.,1.,0.));
#22414=DIRECTION('center_axis',(0.,-1.,0.));
#22415=DIRECTION('ref_axis',(0.528694902398929,0.,-0.848811934516349));
#22416=DIRECTION('center_axis',(0.,-1.,0.));
#22417=DIRECTION('ref_axis',(0.528694902399131,0.,-0.848811934516223));
#22418=DIRECTION('',(0.,1.,0.));
#22419=DIRECTION('center_axis',(0.,1.,0.));
#22420=DIRECTION('ref_axis',(0.528694902399131,0.,-0.848811934516223));
#22421=DIRECTION('center_axis',(0.,-1.,0.));
#22422=DIRECTION('ref_axis',(-0.281918008728675,0.,-0.959438500558769));
#22423=DIRECTION('center_axis',(0.,1.,0.));
#22424=DIRECTION('ref_axis',(-0.281918008754676,0.,-0.959438500551129));
#22425=DIRECTION('',(0.,-1.,0.));
#22426=DIRECTION('center_axis',(0.,-1.,0.));
#22427=DIRECTION('ref_axis',(-0.281918008754676,0.,-0.959438500551129));
#22428=DIRECTION('center_axis',(-0.882269183586981,0.,-0.470745247127108));
#22429=DIRECTION('ref_axis',(-0.470745247127108,0.,0.882269183586981));
#22430=DIRECTION('',(0.470745247127471,0.,-0.882269183586787));
#22431=DIRECTION('',(0.,1.,0.));
#22432=DIRECTION('',(-0.470745247127471,0.,0.882269183586787));
#22433=DIRECTION('center_axis',(0.848811934516349,0.,0.528694902398929));
#22434=DIRECTION('ref_axis',(0.,-1.,0.));
#22435=DIRECTION('',(0.528694902399201,0.,-0.84881193451618));
#22436=DIRECTION('',(0.,-1.,0.));
#22437=DIRECTION('',(-0.528694902399201,0.,0.84881193451618));
#22438=DIRECTION('center_axis',(0.772541698292714,0.,0.634964033941301));
#22439=DIRECTION('ref_axis',(0.,-1.,0.));
#22440=DIRECTION('',(0.634964033941407,0.,-0.772541698292626));
#22441=DIRECTION('',(0.,-1.,0.));
#22442=DIRECTION('',(-0.634964033941407,0.,0.772541698292626));
#22443=DIRECTION('center_axis',(0.581877193327018,0.,0.813276663802591));
#22444=DIRECTION('ref_axis',(0.,-1.,0.));
#22445=DIRECTION('',(0.813276663802457,0.,-0.581877193327205));
#22446=DIRECTION('',(0.,-1.,0.));
#22447=DIRECTION('',(-0.813276663802457,0.,0.581877193327205));
#22448=DIRECTION('center_axis',(0.470745247127107,0.,0.882269183586982));
#22449=DIRECTION('ref_axis',(0.,-1.,0.));
#22450=DIRECTION('',(0.882269183586788,0.,-0.470745247127471));
#22451=DIRECTION('',(0.,-1.,0.));
#22452=DIRECTION('',(-0.882269183586788,0.,0.470745247127471));
#22453=DIRECTION('center_axis',(0.,1.,0.));
#22454=DIRECTION('ref_axis',(-0.902585284349861,0.,0.430511096808295));
#22455=DIRECTION('center_axis',(0.,-1.,0.));
#22456=DIRECTION('ref_axis',(-0.902585284349705,0.,0.430511096808622));
#22457=DIRECTION('',(0.,1.,0.));
#22458=DIRECTION('center_axis',(0.,1.,0.));
#22459=DIRECTION('ref_axis',(-0.902585284349705,0.,0.430511096808622));
#22460=DIRECTION('center_axis',(0.,1.,0.));
#22461=DIRECTION('ref_axis',(-0.902585284349861,0.,0.430511096808295));
#22462=DIRECTION('center_axis',(0.,1.,0.));
#22463=DIRECTION('ref_axis',(-0.902585284349705,0.,0.430511096808622));
#22464=DIRECTION('center_axis',(0.,-1.,0.));
#22465=DIRECTION('ref_axis',(-0.902585284349705,0.,0.430511096808622));
#22466=DIRECTION('center_axis',(0.,1.,0.));
#22467=DIRECTION('ref_axis',(1.,0.,0.));
#22468=DIRECTION('',(0.430511096808718,0.,-0.902585284349659));
#22469=DIRECTION('center_axis',(0.,-1.,0.));
#22470=DIRECTION('ref_axis',(0.902585284349714,0.,-0.430511096808602));
#22471=DIRECTION('',(-0.902585284349657,0.,0.430511096808722));
#22472=DIRECTION('center_axis',(0.,1.,0.));
#22473=DIRECTION('ref_axis',(-0.902585284349705,0.,0.430511096808622));
#22474=DIRECTION('center_axis',(0.,1.,0.));
#22475=DIRECTION('ref_axis',(-0.902585284349705,0.,0.430511096808622));
#22476=DIRECTION('center_axis',(0.,1.,0.));
#22477=DIRECTION('ref_axis',(-0.902585284349705,0.,0.430511096808622));
#22478=DIRECTION('',(0.730368754817616,0.,-0.683053059422301));
#22479=DIRECTION('center_axis',(0.,1.,0.));
#22480=DIRECTION('ref_axis',(-0.902585284349705,0.,0.430511096808622));
#22481=DIRECTION('center_axis',(0.,1.,0.));
#22482=DIRECTION('ref_axis',(-0.902585284349861,0.,0.430511096808295));
#22483=DIRECTION('center_axis',(0.,-1.,0.));
#22484=DIRECTION('ref_axis',(-0.902585284349705,0.,0.430511096808622));
#22485=DIRECTION('',(0.,-1.,0.));
#22486=DIRECTION('center_axis',(0.,1.,0.));
#22487=DIRECTION('ref_axis',(-0.902585284349861,0.,0.430511096808295));
#22488=DIRECTION('',(0.,1.,0.));
#22489=DIRECTION('center_axis',(0.,-1.,0.));
#22490=DIRECTION('ref_axis',(-0.902585284349705,0.,0.430511096808622));
#22491=DIRECTION('center_axis',(0.683053059422266,0.,0.730368754817649));
#22492=DIRECTION('ref_axis',(0.,-1.,0.));
#22493=DIRECTION('',(-0.730368754817616,0.,0.683053059422301));
#22494=DIRECTION('center_axis',(0.,1.,0.));
#22495=DIRECTION('ref_axis',(-0.902585284349861,0.,0.430511096808295));
#22496=DIRECTION('center_axis',(0.,-1.,0.));
#22497=DIRECTION('ref_axis',(-0.902585284349705,0.,0.430511096808622));
#22498=DIRECTION('center_axis',(0.,1.,0.));
#22499=DIRECTION('ref_axis',(0.902585284349861,0.,-0.430511096808295));
#22500=DIRECTION('',(0.,-1.,0.));
#22501=DIRECTION('center_axis',(0.,1.,0.));
#22502=DIRECTION('ref_axis',(0.902585284349714,0.,-0.430511096808602));
#22503=DIRECTION('',(0.,1.,0.));
#22504=DIRECTION('center_axis',(0.430511096808296,0.,0.90258528434986));
#22505=DIRECTION('ref_axis',(0.,-1.,0.));
#22506=DIRECTION('',(0.902585284349657,0.,-0.430511096808722));
#22507=DIRECTION('center_axis',(0.,1.,0.));
#22508=DIRECTION('ref_axis',(-0.902585284349861,0.,0.430511096808295));
#22509=DIRECTION('center_axis',(0.,-1.,0.));
#22510=DIRECTION('ref_axis',(-0.902585284349705,0.,0.430511096808622));
#22511=DIRECTION('center_axis',(-0.902585284349862,0.,-0.430511096808292));
#22512=DIRECTION('ref_axis',(-0.430511096808292,0.,0.902585284349862));
#22513=DIRECTION('',(-0.430511096808718,0.,0.902585284349659));
#22514=DIRECTION('center_axis',(0.,1.,0.));
#22515=DIRECTION('ref_axis',(1.,0.,0.));
#28499=CARTESIAN_POINT('',(0.,0.,0.));
#28500=CARTESIAN_POINT('Origin',(0.0115261780187742,-0.008,-0.00643329000430777));
#28501=CARTESIAN_POINT('',(0.011643864330556,-0.008,-0.00621272270841102));
#28502=CARTESIAN_POINT('',(0.0117444768448874,-0.008,-0.00655513261802572));
#28503=CARTESIAN_POINT('Origin',(0.0115261780187842,-0.00799999999999,-0.00643329000431777));
#28504=CARTESIAN_POINT('',(0.0117444768448874,-0.024,-0.00655513261802572));
#28505=CARTESIAN_POINT('',(0.0117444768448974,-0.00799999999999,-0.00655513261803572));
#28506=CARTESIAN_POINT('',(0.011643864330556,-0.024,-0.00621272270841102));
#28507=CARTESIAN_POINT('Origin',(0.0115261780187842,-0.02400000000001,-0.00643329000431777));
#28508=CARTESIAN_POINT('',(0.011643864330566,-0.00799999999999,-0.00621272270842102));
#28509=CARTESIAN_POINT('Origin',(-4.44089209850063E-17,-0.008,6.72997231505748E-33));
#28510=CARTESIAN_POINT('',(0.0115491497948299,-0.008,-0.00689344899281771));
#28511=CARTESIAN_POINT('Origin',(-4.44089209850063E-17,-0.00799999999999,
6.72997231505748E-33));
#28512=CARTESIAN_POINT('',(0.0115491497948299,-0.024,-0.00689344899281771));
#28513=CARTESIAN_POINT('',(0.0115491497948398,-0.00799999999999,-0.00689344899282771));
#28514=CARTESIAN_POINT('Origin',(-4.44089209850063E-17,-0.02400000000001,
6.72997231505748E-33));
#28515=CARTESIAN_POINT('Origin',(0.0113344815830301,-0.008,-0.00676531797064638));
#28516=CARTESIAN_POINT('',(0.0112023078574304,-0.008,-0.00697752095427546));
#28517=CARTESIAN_POINT('Origin',(0.0113344815830401,-0.00799999999999,-0.00676531797065638));
#28518=CARTESIAN_POINT('',(0.0112023078574304,-0.024,-0.00697752095427546));
#28519=CARTESIAN_POINT('',(0.0112023078574404,-0.00799999999999,-0.00697752095428546));
#28520=CARTESIAN_POINT('Origin',(0.0113344815830401,-0.02400000000001,-0.00676531797065638));
#28521=CARTESIAN_POINT('Origin',(0.0110345551487124,-0.008,-0.00687303373118607));
#28522=CARTESIAN_POINT('',(0.0110345551487124,-0.008,-0.00687303373118607));
#28523=CARTESIAN_POINT('',(0.0108205542946553,-0.00799999999999,-0.00673974017575289));
#28524=CARTESIAN_POINT('',(0.0110345551487124,-0.024,-0.00687303373118607));
#28525=CARTESIAN_POINT('',(0.0110345551487224,-0.016,-0.00687303373119608));
#28526=CARTESIAN_POINT('',(0.0108205542946553,-0.02400000000001,-0.00673974017575289));
#28527=CARTESIAN_POINT('Origin',(0.0105878571202839,-0.008,-0.00788272044413949));
#28528=CARTESIAN_POINT('',(0.0107333264186156,-0.008,-0.00767940127818884));
#28529=CARTESIAN_POINT('',(0.0107883847172589,-0.008,-0.00803201439194517));
#28530=CARTESIAN_POINT('Origin',(0.0105878571202939,-0.00799999999999,-0.00788272044414949));
#28531=CARTESIAN_POINT('',(0.0107883847172589,-0.024,-0.00803201439194517));
#28532=CARTESIAN_POINT('',(0.0107883847172689,-0.00799999999999,-0.00803201439195517));
#28533=CARTESIAN_POINT('',(0.0107333264186156,-0.024,-0.00767940127818884));
#28534=CARTESIAN_POINT('Origin',(0.0105878571202939,-0.02400000000001,-0.00788272044414949));
#28535=CARTESIAN_POINT('',(0.0107333264186256,-0.00799999999999,-0.00767940127819885));
#28536=CARTESIAN_POINT('Origin',(-4.44089209850063E-17,-0.008,6.72997231505748E-33));
#28537=CARTESIAN_POINT('',(0.0105505695690249,-0.008,-0.00834194112716973));
#28538=CARTESIAN_POINT('Origin',(-4.44089209850063E-17,-0.00799999999999,
6.72997231505748E-33));
#28539=CARTESIAN_POINT('',(0.0105505695690249,-0.024,-0.00834194112716973));
#28540=CARTESIAN_POINT('',(0.0105505695690349,-0.00799999999999,-0.00834194112717973));
#28541=CARTESIAN_POINT('Origin',(-4.44089209850063E-17,-0.02400000000001,
6.72997231505748E-33));
#28542=CARTESIAN_POINT('Origin',(0.010354462327965,-0.008,-0.00818688645937847));
#28543=CARTESIAN_POINT('',(0.0101957213194795,-0.008,-0.00838002188395165));
#28544=CARTESIAN_POINT('Origin',(0.010354462327975,-0.00799999999999,-0.00818688645938847));
#28545=CARTESIAN_POINT('',(0.0101957213194795,-0.024,-0.00838002188395165));
#28546=CARTESIAN_POINT('',(0.0101957213194895,-0.00799999999999,-0.00838002188396165));
#28547=CARTESIAN_POINT('Origin',(0.010354462327975,-0.02400000000001,-0.00818688645938847));
#28548=CARTESIAN_POINT('Origin',(0.0100430420778052,-0.008,-0.00825453244123692));
#28549=CARTESIAN_POINT('',(0.0100430420778052,-0.008,-0.00825453244123692));
#28550=CARTESIAN_POINT('',(0.00995338570524485,-0.00799999999999,-0.00818084247458021));
#28551=CARTESIAN_POINT('',(0.0100430420778052,-0.024,-0.00825453244123692));
#28552=CARTESIAN_POINT('',(0.0100430420778153,-0.016,-0.00825453244124692));
#28553=CARTESIAN_POINT('',(0.00995338570524485,-0.02400000000001,-0.00818084247458021));
#28554=CARTESIAN_POINT('Origin',(0.0094683750509568,-0.008,-0.00919727535166899));
#28555=CARTESIAN_POINT('',(0.00963913831581237,-0.008,-0.00901468316296458));
#28556=CARTESIAN_POINT('',(0.0096477003360128,-0.008,-0.00937146617272333));
#28557=CARTESIAN_POINT('Origin',(0.0094683750509668,-0.00799999999999,-0.00919727535167899));
#28558=CARTESIAN_POINT('',(0.0096477003360128,-0.024,-0.00937146617272333));
#28559=CARTESIAN_POINT('',(0.00964770033602281,-0.00799999999999,-0.00937146617273333));
#28560=CARTESIAN_POINT('',(0.00963913831581237,-0.024,-0.00901468316296458));
#28561=CARTESIAN_POINT('Origin',(0.0094683750509668,-0.02400000000001,-0.00919727535167899));
#28562=CARTESIAN_POINT('',(0.00963913831582238,-0.00799999999999,-0.00901468316297458));
#28563=CARTESIAN_POINT('Origin',(-4.44089209850063E-17,-0.008,6.72997231505748E-33));
#28564=CARTESIAN_POINT('',(0.00937146617272329,-0.008,-0.00964770033601285));
#28565=CARTESIAN_POINT('Origin',(-4.44089209850063E-17,-0.00799999999999,
6.72997231505748E-33));
#28566=CARTESIAN_POINT('',(0.00937146617272329,-0.024,-0.00964770033601285));
#28567=CARTESIAN_POINT('',(0.00937146617273328,-0.00799999999999,-0.00964770033602285));
#28568=CARTESIAN_POINT('Origin',(-4.44089209850063E-17,-0.02400000000001,
6.72997231505748E-33));
#28569=CARTESIAN_POINT('Origin',(0.00919727535166896,-0.008,-0.00946837505095685));
#28570=CARTESIAN_POINT('',(0.00901468316296453,-0.008,-0.00963913831581242));
#28571=CARTESIAN_POINT('Origin',(0.00919727535167896,-0.00799999999999,
-0.00946837505096685));
#28572=CARTESIAN_POINT('',(0.00901468316296453,-0.024,-0.00963913831581242));
#28573=CARTESIAN_POINT('',(0.00901468316297454,-0.00799999999999,-0.00963913831582242));
#28574=CARTESIAN_POINT('Origin',(0.00919727535167896,-0.02400000000001,
-0.00946837505096685));
#28575=CARTESIAN_POINT('Origin',(0.00887968977248941,-0.008,-0.00949479381262943));
#28576=CARTESIAN_POINT('',(0.00887968977248941,-0.008,-0.00949479381262943));
#28577=CARTESIAN_POINT('',(0.00881874742507023,-0.00799999999999,-0.00942962993438205));
#28578=CARTESIAN_POINT('',(0.00887968977248941,-0.024,-0.00949479381262943));
#28579=CARTESIAN_POINT('',(0.00887968977249942,-0.016,-0.00949479381263943));
#28580=CARTESIAN_POINT('',(0.00881874742507023,-0.02400000000001,-0.00942962993438205));
#28581=CARTESIAN_POINT('Origin',(0.00818688645937843,-0.008,-0.010354462327965));
#28582=CARTESIAN_POINT('',(0.0083800218839516,-0.008,-0.0101957213194796));
#28583=CARTESIAN_POINT('',(0.00834194112716969,-0.008,-0.0105505695690249));
#28584=CARTESIAN_POINT('Origin',(0.00818688645938842,-0.00799999999999,
-0.010354462327975));
#28585=CARTESIAN_POINT('',(0.00834194112716969,-0.024,-0.0105505695690249));
#28586=CARTESIAN_POINT('',(0.00834194112717969,-0.00799999999999,-0.0105505695690349));
#28587=CARTESIAN_POINT('',(0.0083800218839516,-0.024,-0.0101957213194796));
#28588=CARTESIAN_POINT('Origin',(0.00818688645938842,-0.02400000000001,
-0.010354462327975));
#28589=CARTESIAN_POINT('',(0.00838002188396161,-0.00799999999999,-0.0101957213194896));
#28590=CARTESIAN_POINT('Origin',(-4.44089209850063E-17,-0.008,6.72997231505748E-33));
#28591=CARTESIAN_POINT('',(0.00803201439194512,-0.008,-0.0107883847172589));
#28592=CARTESIAN_POINT('Origin',(-4.44089209850063E-17,-0.00799999999999,
6.72997231505748E-33));
#28593=CARTESIAN_POINT('',(0.00803201439194512,-0.024,-0.0107883847172589));
#28594=CARTESIAN_POINT('',(0.00803201439195512,-0.00799999999999,-0.0107883847172689));
#28595=CARTESIAN_POINT('Origin',(-4.44089209850063E-17,-0.02400000000001,
6.72997231505748E-33));
#28596=CARTESIAN_POINT('Origin',(0.00788272044413945,-0.008,-0.0105878571202839));
#28597=CARTESIAN_POINT('',(0.00767940127818881,-0.008,-0.0107333264186156));
#28598=CARTESIAN_POINT('Origin',(0.00788272044414944,-0.00799999999999,
-0.0105878571202939));
#28599=CARTESIAN_POINT('',(0.00767940127818881,-0.024,-0.0107333264186156));
#28600=CARTESIAN_POINT('',(0.00767940127819881,-0.00799999999999,-0.0107333264186256));
#28601=CARTESIAN_POINT('Origin',(0.00788272044414944,-0.02400000000001,
-0.0105878571202939));
#28602=CARTESIAN_POINT('Origin',(0.00756440351325119,-0.008,-0.0105725966294337));
#28603=CARTESIAN_POINT('',(0.00756440351325119,-0.008,-0.0105725966294337));
#28604=CARTESIAN_POINT('',(0.00746427554955173,-0.00799999999999,-0.0104326500269426));
#28605=CARTESIAN_POINT('',(0.00756440351325119,-0.024,-0.0105725966294337));
#28606=CARTESIAN_POINT('',(0.00756440351326119,-0.016,-0.0105725966294437));
#28607=CARTESIAN_POINT('',(0.00746427554955173,-0.02400000000001,-0.0104326500269426));
#28608=CARTESIAN_POINT('Origin',(0.00676531797064634,-0.008,-0.0113344815830301));
#28609=CARTESIAN_POINT('',(0.00697752095427543,-0.008,-0.0112023078574304));
#28610=CARTESIAN_POINT('',(0.00689344899281767,-0.008,-0.0115491497948299));
#28611=CARTESIAN_POINT('Origin',(0.00676531797065634,-0.00799999999999,
-0.0113344815830401));
#28612=CARTESIAN_POINT('',(0.00689344899281767,-0.024,-0.0115491497948299));
#28613=CARTESIAN_POINT('',(0.00689344899282767,-0.00799999999999,-0.0115491497948399));
#28614=CARTESIAN_POINT('',(0.00697752095427543,-0.024,-0.0112023078574304));
#28615=CARTESIAN_POINT('Origin',(0.00676531797065634,-0.02400000000001,
-0.0113344815830401));
#28616=CARTESIAN_POINT('',(0.00697752095428543,-0.00799999999999,-0.0112023078574404));
#28617=CARTESIAN_POINT('Origin',(-4.44089209850063E-17,-0.008,6.72997231505748E-33));
#28618=CARTESIAN_POINT('',(0.00655513261802568,-0.008,-0.0117444768448874));
#28619=CARTESIAN_POINT('Origin',(-4.44089209850063E-17,-0.00799999999999,
6.72997231505748E-33));
#28620=CARTESIAN_POINT('',(0.00655513261802568,-0.024,-0.0117444768448874));
#28621=CARTESIAN_POINT('',(0.00655513261803568,-0.00799999999999,-0.0117444768448974));
#28622=CARTESIAN_POINT('Origin',(-4.44089209850063E-17,-0.02400000000001,
6.72997231505748E-33));
#28623=CARTESIAN_POINT('Origin',(0.00643329000430773,-0.008,-0.0115261780187742));
#28624=CARTESIAN_POINT('',(0.00621272270841099,-0.008,-0.011643864330556));
#28625=CARTESIAN_POINT('Origin',(0.00643329000431773,-0.00799999999999,
-0.0115261780187842));
#28626=CARTESIAN_POINT('',(0.00621272270841099,-0.024,-0.011643864330556));
#28627=CARTESIAN_POINT('',(0.00621272270842099,-0.00799999999999,-0.011643864330566));
#28628=CARTESIAN_POINT('Origin',(0.00643329000431773,-0.02400000000001,
-0.0115261780187842));
#28629=CARTESIAN_POINT('Origin',(0.00611968821265236,-0.008,-0.0114694993866308));
#28630=CARTESIAN_POINT('',(0.00611968821265236,-0.008,-0.0114694993866308));
#28631=CARTESIAN_POINT('',(0.00594871026243935,-0.00799999999999,-0.0111490530784194));
#28632=CARTESIAN_POINT('',(0.00611968821265236,-0.024,-0.0114694993866308));
#28633=CARTESIAN_POINT('',(0.00611968821266236,-0.016,-0.0114694993866408));
#28634=CARTESIAN_POINT('',(0.00594871026243935,-0.02400000000001,-0.0111490530784194));
#28635=CARTESIAN_POINT('Origin',(0.00711094643726556,-0.008,-0.0114165205192449));
#28636=CARTESIAN_POINT('',(0.00687303373118604,-0.024,-0.0110345551487125));
#28637=CARTESIAN_POINT('',(0.00685869652879261,-0.02400000000001,-0.0110115369799216));
#28638=CARTESIAN_POINT('',(0.00687303373118604,-0.008,-0.0110345551487125));
#28639=CARTESIAN_POINT('',(0.00687303373119604,-0.016,-0.0110345551487225));
#28640=CARTESIAN_POINT('',(0.00685869652879261,-0.00799999999999,-0.0110115369799216));
#28641=CARTESIAN_POINT('Origin',(0.00854026625651046,-0.008,-0.010390685842037));
#28642=CARTESIAN_POINT('',(0.00825453244123687,-0.024,-0.0100430420778053));
#28643=CARTESIAN_POINT('',(0.00832370938221696,-0.02400000000001,-0.0101272075873608));
#28644=CARTESIAN_POINT('',(0.00825453244123687,-0.008,-0.0100430420778053));
#28645=CARTESIAN_POINT('',(0.00825453244124687,-0.016,-0.0100430420778153));
#28646=CARTESIAN_POINT('',(0.00832370938221696,-0.00799999999999,-0.0101272075873608));
#28647=CARTESIAN_POINT('Origin',(0.0109385711281449,-0.008,-0.00782624825024839));
#28648=CARTESIAN_POINT('',(0.0105725966294337,-0.024,-0.00756440351325123));
#28649=CARTESIAN_POINT('',(0.0106156372762982,-0.02400000000001,-0.00759519791805035));
#28650=CARTESIAN_POINT('',(0.0105725966294337,-0.008,-0.00756440351325123));
#28651=CARTESIAN_POINT('',(0.0105725966294436,-0.016,-0.00756440351326123));
#28652=CARTESIAN_POINT('',(0.0106156372762982,-0.00799999999999,-0.00759519791805035));
#28653=CARTESIAN_POINT('Origin',(0.0118665205192449,-0.008,-0.0063315235738596));
#28654=CARTESIAN_POINT('',(0.0114694993866308,-0.024,-0.0061196882126524));
#28655=CARTESIAN_POINT('',(0.0113475636447265,-0.02400000000001,-0.00605462794304299));
#28656=CARTESIAN_POINT('',(0.0114694993866308,-0.008,-0.0061196882126524));
#28657=CARTESIAN_POINT('',(0.0114694993866408,-0.016,-0.0061196882126624));
#28658=CARTESIAN_POINT('',(0.0113475636447265,-0.00799999999999,-0.00605462794304299));
#28659=CARTESIAN_POINT('Origin',(-4.44089209850063E-17,-0.016,6.72997231505748E-33));
#28660=CARTESIAN_POINT('',(0.0055966442585078,-0.008,-0.0117336086965482));
#28661=CARTESIAN_POINT('Origin',(-4.44089209850063E-17,-0.00799999999999,
6.72997231505748E-33));
#28662=CARTESIAN_POINT('',(0.0055966442585078,-0.024,-0.0117336086965482));
#28663=CARTESIAN_POINT('',(0.0055966442585178,-0.016,-0.0117336086965582));
#28664=CARTESIAN_POINT('Origin',(-4.44089209850063E-17,-0.02400000000001,
6.72997231505748E-33));
#28665=CARTESIAN_POINT('Origin',(-4.44089209850063E-17,-0.016,6.72997231505748E-33));
#28666=CARTESIAN_POINT('Origin',(-4.44089209850063E-17,-0.02400000000001,
6.72997231505748E-33));
#28667=CARTESIAN_POINT('Origin',(-4.44089209850063E-17,-0.00799999999999,
6.72997231505748E-33));
#28668=CARTESIAN_POINT('Origin',(0.00907128985548541,-0.024,-0.00907128985548545));
#28669=CARTESIAN_POINT('',(0.00598410424563526,-0.024,-0.0125459354524631));
#28670=CARTESIAN_POINT('',(0.00598410424564526,-0.02400000000001,-0.0125459354524731));
#28671=CARTESIAN_POINT('',(0.0125459354524631,-0.024,-0.0059841042456353));
#28672=CARTESIAN_POINT('Origin',(-4.44089209850063E-17,-0.02400000000001,
6.72997231505748E-33));
#28673=CARTESIAN_POINT('',(0.0117336086965482,-0.024,-0.00559664425850784));
#28674=CARTESIAN_POINT('',(0.0117336086965582,-0.02400000000001,-0.00559664425851784));
#28675=CARTESIAN_POINT('Origin',(-4.44089209850063E-17,-0.02400000000001,
6.72997231505748E-33));
#28676=CARTESIAN_POINT('Origin',(-4.44089209850063E-17,-0.02400000000001,
6.72997231505748E-33));
#28677=CARTESIAN_POINT('',(0.00949479381262939,-0.024,-0.00887968977248946));
#28678=CARTESIAN_POINT('Origin',(-4.44089209850063E-17,-0.02400000000001,
6.72997231505748E-33));
#28679=CARTESIAN_POINT('',(0.00959396290421598,-0.02400000000001,-0.00897243436344028));
#28680=CARTESIAN_POINT('Origin',(-4.44089209850063E-17,-0.02400000000001,
6.72997231505748E-33));
#28681=CARTESIAN_POINT('Origin',(-4.44089209850063E-17,-0.016,6.72997231505748E-33));
#28682=CARTESIAN_POINT('',(0.00949479381262939,-0.008,-0.00887968977248946));
#28683=CARTESIAN_POINT('Origin',(-4.44089209850063E-17,-0.00799999999999,
6.72997231505748E-33));
#28684=CARTESIAN_POINT('',(0.00949479381263939,-0.016,-0.00887968977249946));
#28685=CARTESIAN_POINT('Origin',(-4.44089209850063E-17,-0.016,6.72997231505748E-33));
#28686=CARTESIAN_POINT('',(0.0117336086965482,-0.008,-0.00559664425850784));
#28687=CARTESIAN_POINT('',(0.0117336086965582,-0.016,-0.00559664425851784));
#28688=CARTESIAN_POINT('Origin',(-4.44089209850063E-17,-0.00799999999999,
6.72997231505748E-33));
#28689=CARTESIAN_POINT('Origin',(0.00982345975229732,-0.008,-0.00918706364922948));
#28690=CARTESIAN_POINT('',(0.00959396290421598,-0.00799999999999,-0.00897243436344028));
#28691=CARTESIAN_POINT('Origin',(-4.44089209850063E-17,-0.016,6.72997231505748E-33));
#28692=CARTESIAN_POINT('Origin',(-4.44089209850063E-17,-0.00799999999999,
6.72997231505748E-33));
#28693=CARTESIAN_POINT('Origin',(-4.44089209850063E-17,-0.016,6.72997231505748E-33));
#28694=CARTESIAN_POINT('',(0.00598410424563526,-0.008,-0.0125459354524631));
#28695=CARTESIAN_POINT('',(0.00598410424564526,-0.016,-0.0125459354524731));
#28696=CARTESIAN_POINT('',(0.0125459354524631,-0.008,-0.0059841042456353));
#28697=CARTESIAN_POINT('Origin',(-4.44089209850063E-17,-0.00799999999999,
6.72997231505748E-33));
#28698=CARTESIAN_POINT('',(0.0125459354524731,-0.016,-0.0059841042456453));
#28699=CARTESIAN_POINT('Origin',(0.0117336086965482,-0.016,-0.00559664425850784));
#28700=CARTESIAN_POINT('',(0.0117336086965582,-0.00799999999999,-0.00559664425851784));
#28701=CARTESIAN_POINT('Origin',(-4.44089209850063E-17,-0.016,6.72997231505748E-33));
#28702=CARTESIAN_POINT('Origin',(-4.44089209850063E-17,-0.00799999999999,
6.72997231505748E-33));
#28703=CARTESIAN_POINT('Origin',(0.00598410424563526,-0.016,-0.0125459354524631));
#28704=CARTESIAN_POINT('',(0.00598410424564526,-0.00799999999999,-0.0125459354524731));
#28705=CARTESIAN_POINT('Origin',(0.00907128985548541,-0.008,-0.00907128985548545));
#34809=UNCERTAINTY_MEASURE_WITH_UNIT(LENGTH_MEASURE(1.E-5),#34877,
'DISTANCE_ACCURACY_VALUE',
'Maximum model space distance between geometric entities at asserted c
onnectivities');
#34841=UNCERTAINTY_MEASURE_WITH_UNIT(LENGTH_MEASURE(1.E-5),#34877,
'DISTANCE_ACCURACY_VALUE',
'Maximum model space distance between geometric entities at asserted c
onnectivities');
#34844=(
GEOMETRIC_REPRESENTATION_CONTEXT(3)
GLOBAL_UNCERTAINTY_ASSIGNED_CONTEXT((#34809))
GLOBAL_UNIT_ASSIGNED_CONTEXT((#34877,#34878,#34879))
REPRESENTATION_CONTEXT('','3D')
);
#34876=(
GEOMETRIC_REPRESENTATION_CONTEXT(3)
GLOBAL_UNCERTAINTY_ASSIGNED_CONTEXT((#34841))
GLOBAL_UNIT_ASSIGNED_CONTEXT((#34877,#34878,#34879))
REPRESENTATION_CONTEXT('','3D')
);
#34877=(
LENGTH_UNIT()
NAMED_UNIT(*)
SI_UNIT($,.METRE.)
);
#34878=(
NAMED_UNIT(*)
PLANE_ANGLE_UNIT()
SI_UNIT($,.RADIAN.)
);
#34879=(
NAMED_UNIT(*)
SI_UNIT($,.STERADIAN.)
SOLID_ANGLE_UNIT()
);
#34882=SHAPE_DEFINITION_REPRESENTATION(#34916,#34986);
#34916=PRODUCT_DEFINITION_SHAPE('',$,#35021);
#34986=SHAPE_REPRESENTATION('',(#19969),#34844);
#35018=PRODUCT_DEFINITION_CONTEXT('part definition',#35122,'design');
#35021=PRODUCT_DEFINITION('Motor Stator Face 1','Motor Stator Face 1',#35055,
#35018);
#35055=PRODUCT_DEFINITION_FORMATION('',$,#35126);
#35122=APPLICATION_CONTEXT('Managed model based 3d engineering');
#35123=PRODUCT_CONTEXT('part definition',#35122,'mechanical');
#35126=PRODUCT('Motor Stator Face 1','Motor Stator Face 1',
'LEGAL AND USAGE DISCLAIMER: this Data/Model is provided \X2\201C\X0\A
S IS\X2\201D\X0\ for informational and representational only. It is a 
geometric approximation and is NOT engineered, certified, or guarantee
d for dimensional accuracy, exact tolerances, or production-level prec
ision. Vendor disclaims all implied warranties including fitness for a
 particular purpose. DO NOT USE FOR DIRECT PHYSICAL MANUFACTURING, AUT
OMATED PRODUCTION, OR SAFETY-CRITICAL SYSTEMS without independent engi
neering verification and resolution of any design discrepancies.',(#35123));
#35160=PRESENTATION_STYLE_ASSIGNMENT((#35169));
#35169=SURFACE_STYLE_USAGE(.BOTH.,#35178);
#35178=SURFACE_SIDE_STYLE('',(#35187));
#35187=SURFACE_STYLE_FILL_AREA(#35196);
#35196=FILL_AREA_STYLE('Plastic - Glossy (Black)',(#35205));
#35205=FILL_AREA_STYLE_COLOUR('Plastic - Glossy (Black)',#35214);
#35214=COLOUR_RGB('Plastic - Glossy (Black)',0.0980392156862745,0.0980392156862745,
0.0980392156862745);
ENDSEC;
END-ISO-10303-21;
